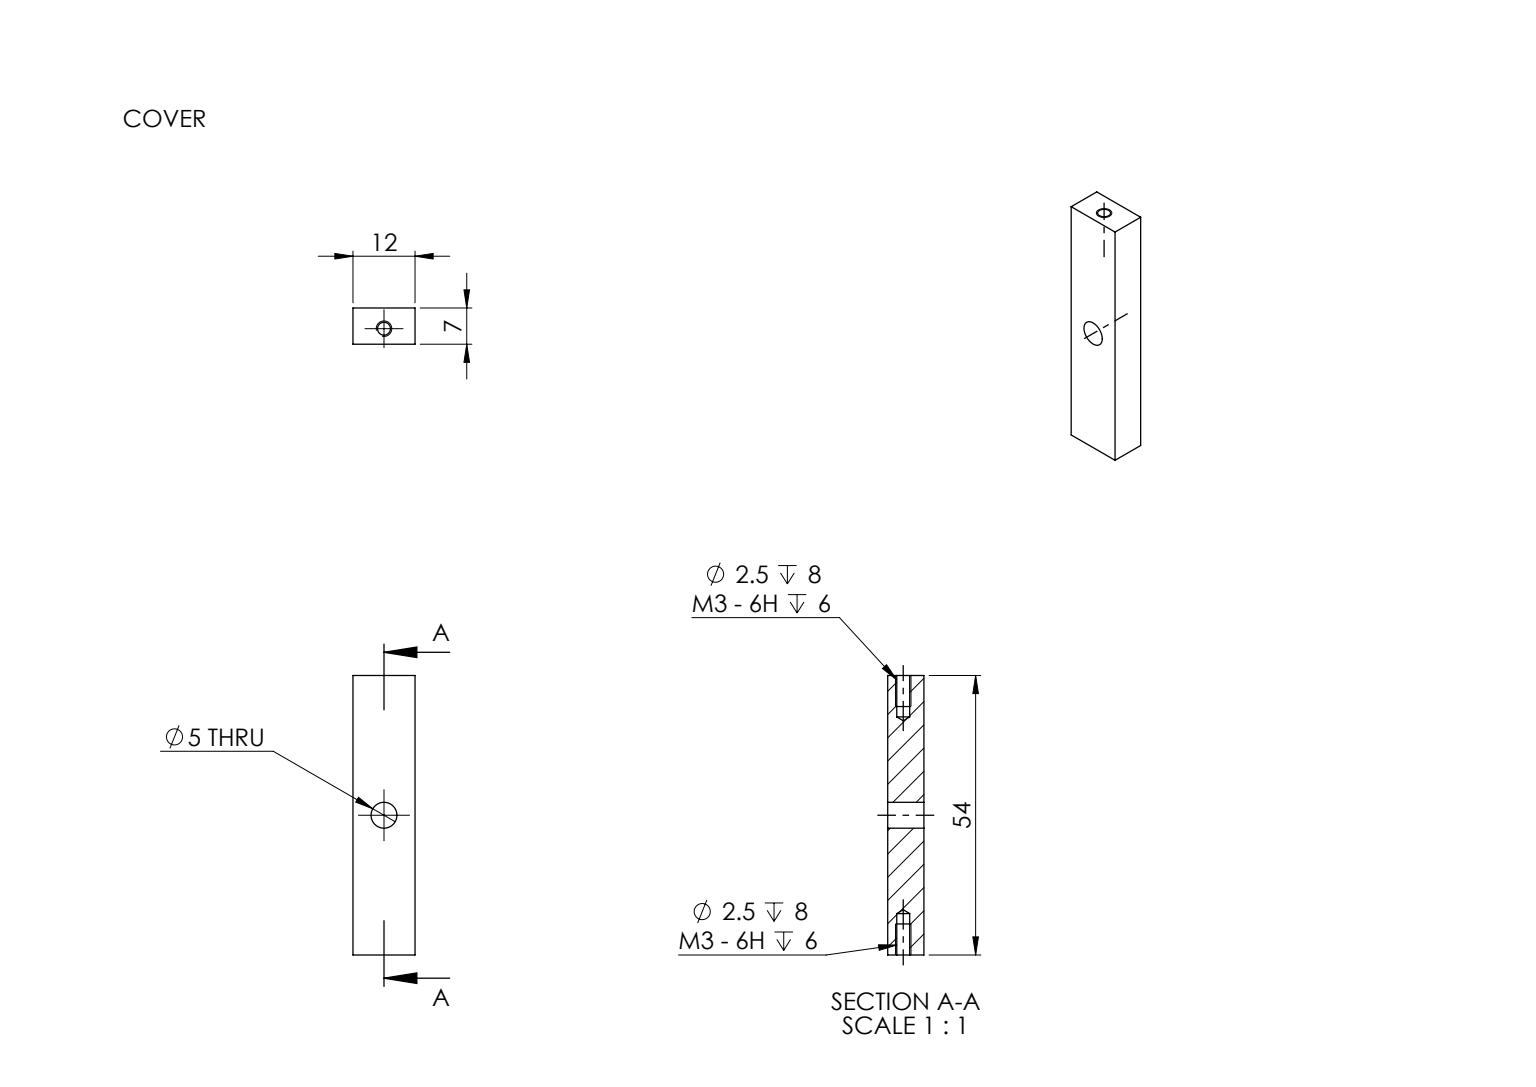
ISO-10303-21;
HEADER;
FILE_DESCRIPTION (('STEP AP214'),
    '1' );
FILE_NAME ('cover.step',
    '2026-10-03T18:28:46',
    ( '' ),
    ( '' ),
    'SwSTEP 2.0',
    'SolidWorks 2026',
    '' );
FILE_SCHEMA (( 'AUTOMOTIVE_DESIGN' ));
ENDSEC;

DATA;
#4=DIRECTION ( 'NONE',  ( 0.000000000000000000, 0.000000000000000000, 1.000000000000000000 ) ) ;
#12=PLANE ( 'NONE',  #9677 ) ;
#144=VERTEX_POINT ( 'NONE', #4838 ) ;
#200=CARTESIAN_POINT ( 'NONE',  ( 1.530808498934188612E-16, 18.99999999999999289, -1.249999999999997558 ) ) ;
#299=( NAMED_UNIT ( * ) SI_UNIT ( $, .STERADIAN. ) SOLID_ANGLE_UNIT ( ) );
#306=FACE_BOUND ( 'NONE', #5426, .T. ) ;
#314=ORIENTED_EDGE ( 'NONE', *, *, #8184, .T. ) ;
#318=DIRECTION ( 'NONE',  ( -0.000000000000000000, -1.000000000000000000, -0.000000000000000000 ) ) ;
#340=ADVANCED_FACE ( 'NONE', ( #9129 ), #3510, .F. ) ;
#376=VERTEX_POINT ( 'NONE', #586 ) ;
#381=DIRECTION ( 'NONE',  ( 1.000000000000000000, 0.000000000000000000, 0.000000000000000000 ) ) ;
#393=CARTESIAN_POINT ( 'NONE',  ( 5.999999999999999112, -27.00000000000000711, -4.000000000000000000 ) ) ;
#434=VECTOR ( 'NONE', #3012, 1000.000000000000000 ) ;
#442=CONICAL_SURFACE ( 'NONE', #7548, 1.249999999999997558, 1.029744258676650981 ) ;
#476=ORIENTED_EDGE ( 'NONE', *, *, #8711, .T. ) ;
#479=LINE ( 'NONE', #8439, #7690 ) ;
#491=LINE ( 'NONE', #2876, #2720 ) ;
#505=VERTEX_POINT ( 'NONE', #7751 ) ;
#514=AXIS2_PLACEMENT_3D ( 'NONE', #1323, #4706, #9556 ) ;
#518=LINE ( 'NONE', #5183, #846 ) ;
#555=ORIENTED_EDGE ( 'NONE', *, *, #4207, .T. ) ;
#586=CARTESIAN_POINT ( 'NONE',  ( 5.999999999999999112, -27.00000000000000711, 3.000000000000000000 ) ) ;
#608=AXIS2_PLACEMENT_3D ( 'NONE', #7258, #8118, #4082 ) ;
#678=CARTESIAN_POINT ( 'NONE',  ( -5.999999999999999112, 26.99999999999999289, 3.000000000000000000 ) ) ;
#712=EDGE_CURVE ( 'NONE', #980, #3093, #750, .T. ) ;
#736=ADVANCED_FACE ( 'NONE', ( #5713 ), #5223, .F. ) ;
#745=DIRECTION ( 'NONE',  ( 0.000000000000000000, 0.000000000000000000, -1.000000000000000000 ) ) ;
#750=LINE ( 'NONE', #3983, #6059 ) ;
#753=FACE_OUTER_BOUND ( 'NONE', #4033, .T. ) ;
#759=DIRECTION ( 'NONE',  ( 0.000000000000000000, 0.000000000000000000, 1.000000000000000000 ) ) ;
#766=VECTOR ( 'NONE', #8542, 1000.000000000000000 ) ;
#808=EDGE_CURVE ( 'NONE', #505, #2310, #6880, .T. ) ;
#822=CARTESIAN_POINT ( 'NONE',  ( 5.999999999999999112, -27.00000000000000711, 3.000000000000000000 ) ) ;
#823=LINE ( 'NONE', #9950, #1369 ) ;
#832=( NAMED_UNIT ( * ) SI_UNIT ( $, .STERADIAN. ) SOLID_ANGLE_UNIT ( ) );
#846=VECTOR ( 'NONE', #2165, 1000.000000000000000 ) ;
#851=DIRECTION ( 'NONE',  ( 1.000000000000000000, 0.000000000000000000, -0.000000000000000000 ) ) ;
#854=DIRECTION ( 'NONE',  ( -0.000000000000000000, -1.000000000000000000, -0.000000000000000000 ) ) ;
#856=ADVANCED_FACE ( 'NONE', ( #9639 ), #6825, .F. ) ;
#881=ORIENTED_EDGE ( 'NONE', *, *, #2871, .T. ) ;
#893=ORIENTED_EDGE ( 'NONE', *, *, #4207, .F. ) ;
#945=CARTESIAN_POINT ( 'NONE',  ( 5.999999999999999112, -27.00000000000000711, 3.000000000000000000 ) ) ;
#954=ORIENTED_EDGE ( 'NONE', *, *, #7254, .T. ) ;
#959=DIRECTION ( 'NONE',  ( 0.000000000000000000, 0.000000000000000000, 1.000000000000000000 ) ) ;
#968=DIRECTION ( 'NONE',  ( 0.000000000000000000, -0.000000000000000000, 1.000000000000000000 ) ) ;
#980=VERTEX_POINT ( 'NONE', #1783 ) ;
#999=AXIS2_PLACEMENT_3D ( 'NONE', #8960, #854, #1703 ) ;
#1002=LINE ( 'NONE', #6167, #3911 ) ;
#1048=DIRECTION ( 'NONE',  ( 0.000000000000000000, 0.000000000000000000, 1.000000000000000000 ) ) ;
#1072=CARTESIAN_POINT ( 'NONE',  ( 0.000000000000000000, 0.000000000000000000, 3.000000000000000000 ) ) ;
#1082=DIRECTION ( 'NONE',  ( 0.000000000000000000, 0.000000000000000000, 1.000000000000000000 ) ) ;
#1092=ORIENTED_EDGE ( 'NONE', *, *, #2254, .T. ) ;
#1117=ADVANCED_FACE ( 'NONE', ( #3941 ), #1519, .F. ) ;
#1213=FACE_OUTER_BOUND ( 'NONE', #9376, .T. ) ;
#1232=ADVANCED_FACE ( 'NONE', ( #4199 ), #9733, .F. ) ;
#1248=VERTEX_POINT ( 'NONE', #9686 ) ;
#1263=COLOUR_RGB ( '', 0.08235294, 0.09019608, 0.10196078) ;
#1265=ORIENTED_EDGE ( 'NONE', *, *, #6212, .T. ) ;
#1287=DIRECTION ( 'NONE',  ( -0.000000000000000000, 1.000000000000000000, -0.000000000000000000 ) ) ;
#1323=CARTESIAN_POINT ( 'NONE',  ( 0.000000000000000000, -27.00000000000000711, 0.000000000000000000 ) ) ;
#1331=EDGE_LOOP ( 'NONE', ( #6517, #9789, #7113 ) ) ;
#1334=LINE ( 'NONE', #10258, #2894 ) ;
#1349=VERTEX_POINT ( 'NONE', #6518 ) ;
#1351=AXIS2_PLACEMENT_3D ( 'NONE', #4874, #3979, #851 ) ;
#1359=ORIENTED_EDGE ( 'NONE', *, *, #6212, .F. ) ;
#1363=ADVANCED_FACE ( 'NONE', ( #2503, #753 ), #12, .F. ) ;
#1369=VECTOR ( 'NONE', #9141, 1000.000000000000000 ) ;
#1410=EDGE_LOOP ( 'NONE', ( #9527, #2908, #2491, #4743 ) ) ;
#1428=CARTESIAN_POINT ( 'NONE',  ( 1.530808498934183189E-16, 26.99999999999999289, -1.249999999999993339 ) ) ;
#1447=CARTESIAN_POINT ( 'NONE',  ( 0.000000000000000000, -19.00000000000000711, 0.000000000000000000 ) ) ;
#1448=CARTESIAN_POINT ( 'NONE',  ( 0.000000000000000000, 0.000000000000000000, -4.000000000000000000 ) ) ;
#1484=PRODUCT_DEFINITION_SHAPE ( 'NONE', 'NONE',  #7235 ) ;
#1488=DIRECTION ( 'NONE',  ( 0.000000000000000000, 0.000000000000000000, -1.000000000000000000 ) ) ;
#1517=EDGE_LOOP ( 'NONE', ( #6768, #8667, #1604, #8725 ) ) ;
#1519=CONICAL_SURFACE ( 'NONE', #7440, 1.249999999999997558, 1.029744258676650981 ) ;
#1523=CIRCLE ( 'NONE', #5067, 1.249999999999997558 ) ;
#1536=ORIENTED_EDGE ( 'NONE', *, *, #808, .F. ) ;
#1604=ORIENTED_EDGE ( 'NONE', *, *, #5366, .F. ) ;
#1610=CARTESIAN_POINT ( 'NONE',  ( 0.000000000000000000, 26.99999999999999289, 0.000000000000000000 ) ) ;
#1636=CARTESIAN_POINT ( 'NONE',  ( 0.000000000000000000, -19.00000000000000711, 0.000000000000000000 ) ) ;
#1648=CARTESIAN_POINT ( 'NONE',  ( -2.500000000000000000, 0.000000000000000000, -4.000000000000000000 ) ) ;
#1703=DIRECTION ( 'NONE',  ( 0.000000000000000000, 0.000000000000000000, -1.000000000000000000 ) ) ;
#1749=CARTESIAN_POINT ( 'NONE',  ( -5.999999999999999112, -27.00000000000000711, 3.000000000000000000 ) ) ;
#1760=CARTESIAN_POINT ( 'NONE',  ( -2.143395387092215042E-15, 18.24892422621553933, 0.000000000000000000 ) ) ;
#1776=STYLED_ITEM ( 'NONE', ( #2430 ), #4603 ) ;
#1783=CARTESIAN_POINT ( 'NONE',  ( 0.000000000000000000, -19.00000000000000711, -1.249999999999997558 ) ) ;
#1802=VERTEX_POINT ( 'NONE', #4484 ) ;
#1843=DIRECTION ( 'NONE',  ( -0.000000000000000000, -0.000000000000000000, -1.000000000000000000 ) ) ;
#1857=EDGE_LOOP ( 'NONE', ( #8302, #4110, #3466, #8986 ) ) ;
#1921=AXIS2_PLACEMENT_3D ( 'NONE', #4104, #7391, #9842 ) ;
#1938=SURFACE_SIDE_STYLE ('',( #5055 ) ) ;
#1940=DIRECTION ( 'NONE',  ( 1.049727191138616477E-16, 0.5150380749100571531, -0.8571673007021105573 ) ) ;
#1984=VERTEX_POINT ( 'NONE', #3956 ) ;
#2012=DIRECTION ( 'NONE',  ( 0.000000000000000000, 0.000000000000000000, -1.000000000000000000 ) ) ;
#2039=EDGE_CURVE ( 'NONE', #10462, #144, #1334, .T. ) ;
#2047=AXIS2_PLACEMENT_3D ( 'NONE', #4230, #7668, #6862 ) ;
#2059=ORIENTED_EDGE ( 'NONE', *, *, #712, .F. ) ;
#2087=DIRECTION ( 'NONE',  ( 0.000000000000000000, 0.000000000000000000, 1.000000000000000000 ) ) ;
#2092=ORIENTED_EDGE ( 'NONE', *, *, #8374, .F. ) ;
#2101=AXIS2_PLACEMENT_3D ( 'NONE', #7090, #5610, #4547 ) ;
#2107=ORIENTED_EDGE ( 'NONE', *, *, #2498, .F. ) ;
#2151=ORIENTED_EDGE ( 'NONE', *, *, #8374, .T. ) ;
#2165=DIRECTION ( 'NONE',  ( 0.000000000000000000, 0.5150380749100571531, 0.8571673007021105573 ) ) ;
#2185=EDGE_CURVE ( 'NONE', #2333, #7985, #10306, .T. ) ;
#2188=CYLINDRICAL_SURFACE ( 'NONE', #3728, 1.249999999999993339 ) ;
#2191=AXIS2_PLACEMENT_3D ( 'NONE', #9273, #3497, #2012 ) ;
#2198=AXIS2_PLACEMENT_3D ( 'NONE', #6512, #3925, #1488 ) ;
#2204=VECTOR ( 'NONE', #5118, 1000.000000000000000 ) ;
#2216=ORIENTED_EDGE ( 'NONE', *, *, #7634, .T. ) ;
#2254=EDGE_CURVE ( 'NONE', #2333, #3169, #4079, .T. ) ;
#2291=ADVANCED_FACE ( 'NONE', ( #10464 ), #5710, .F. ) ;
#2310=VERTEX_POINT ( 'NONE', #1648 ) ;
#2332=CARTESIAN_POINT ( 'NONE',  ( 5.999999999999999112, 26.99999999999999289, -4.000000000000000000 ) ) ;
#2333=VERTEX_POINT ( 'NONE', #9816 ) ;
#2368=CIRCLE ( 'NONE', #2191, 1.249999999999988898 ) ;
#2382=AXIS2_PLACEMENT_3D ( 'NONE', #945, #5065, #1048 ) ;
#2430=PRESENTATION_STYLE_ASSIGNMENT (( #9052 ) ) ;
#2450=DIRECTION ( 'NONE',  ( -0.000000000000000000, -1.000000000000000000, -0.000000000000000000 ) ) ;
#2464=ADVANCED_FACE ( 'NONE', ( #4525 ), #8276, .F. ) ;
#2471=ORIENTED_EDGE ( 'NONE', *, *, #4014, .F. ) ;
#2491=ORIENTED_EDGE ( 'NONE', *, *, #9814, .T. ) ;
#2498=EDGE_CURVE ( 'NONE', #1349, #2589, #1002, .T. ) ;
#2503=FACE_BOUND ( 'NONE', #5490, .T. ) ;
#2529=FILL_AREA_STYLE_COLOUR ( '', #1263 ) ;
#2585=EDGE_LOOP ( 'NONE', ( #7497, #6215 ) ) ;
#2589=VERTEX_POINT ( 'NONE', #3684 ) ;
#2638=CARTESIAN_POINT ( 'NONE',  ( 1.530808498934183189E-16, -27.00000000000000711, 1.249999999999993339 ) ) ;
#2639=ORIENTED_EDGE ( 'NONE', *, *, #5366, .T. ) ;
#2673=EDGE_CURVE ( 'NONE', #376, #8882, #4052, .T. ) ;
#2684=ORIENTED_EDGE ( 'NONE', *, *, #6082, .F. ) ;
#2699=CARTESIAN_POINT ( 'NONE',  ( 1.530808498934180724E-16, 26.99999999999999289, -1.249999999999988898 ) ) ;
#2720=VECTOR ( 'NONE', #5313, 1000.000000000000000 ) ;
#2732=( NAMED_UNIT ( * ) PLANE_ANGLE_UNIT ( ) SI_UNIT ( $, .RADIAN. ) );
#2738=VERTEX_POINT ( 'NONE', #4684 ) ;
#2765=DIRECTION ( 'NONE',  ( 0.000000000000000000, 0.000000000000000000, 1.000000000000000000 ) ) ;
#2782=( LENGTH_UNIT ( ) NAMED_UNIT ( * ) SI_UNIT ( .MILLI., .METRE. ) );
#2827=FACE_OUTER_BOUND ( 'NONE', #1857, .T. ) ;
#2829=LINE ( 'NONE', #393, #4246 ) ;
#2851=CARTESIAN_POINT ( 'NONE',  ( 0.000000000000000000, 18.99999999999999289, 0.000000000000000000 ) ) ;
#2871=EDGE_CURVE ( 'NONE', #2310, #2589, #6449, .T. ) ;
#2876=CARTESIAN_POINT ( 'NONE',  ( 5.999999999999999112, -27.00000000000000711, 3.000000000000000000 ) ) ;
#2889=VECTOR ( 'NONE', #6206, 1000.000000000000000 ) ;
#2894=VECTOR ( 'NONE', #9353, 1000.000000000000000 ) ;
#2908=ORIENTED_EDGE ( 'NONE', *, *, #10395, .T. ) ;
#2936=DIRECTION ( 'NONE',  ( 1.000000000000000000, -0.000000000000000000, -0.000000000000000000 ) ) ;
#2937=EDGE_CURVE ( 'NONE', #9930, #8882, #2829, .T. ) ;
#2975=CYLINDRICAL_SURFACE ( 'NONE', #514, 1.249999999999993339 ) ;
#3012=DIRECTION ( 'NONE',  ( -0.000000000000000000, -1.000000000000000000, -0.000000000000000000 ) ) ;
#3013=DIRECTION ( 'NONE',  ( 0.000000000000000000, 0.000000000000000000, 1.000000000000000000 ) ) ;
#3067=ORIENTED_EDGE ( 'NONE', *, *, #6295, .F. ) ;
#3085=CARTESIAN_POINT ( 'NONE',  ( -5.999999999999999112, -27.00000000000000711, -4.000000000000000000 ) ) ;
#3093=VERTEX_POINT ( 'NONE', #6105 ) ;
#3165=( NAMED_UNIT ( * ) PLANE_ANGLE_UNIT ( ) SI_UNIT ( $, .RADIAN. ) );
#3169=VERTEX_POINT ( 'NONE', #4725 ) ;
#3236=FACE_OUTER_BOUND ( 'NONE', #4534, .T. ) ;
#3242=DIRECTION ( 'NONE',  ( 0.000000000000000000, -1.000000000000000000, 0.000000000000000000 ) ) ;
#3246=PRODUCT_CONTEXT ( 'NONE', #3297, 'mechanical' ) ;
#3254=CARTESIAN_POINT ( 'NONE',  ( -5.999999999999999112, -27.00000000000000711, 3.000000000000000000 ) ) ;
#3262=EDGE_LOOP ( 'NONE', ( #4954, #10176, #7125, #4590 ) ) ;
#3297=APPLICATION_CONTEXT ( 'automotive_design' ) ;
#3321=ADVANCED_FACE ( 'NONE', ( #3774 ), #442, .F. ) ;
#3466=ORIENTED_EDGE ( 'NONE', *, *, #2185, .T. ) ;
#3496=EDGE_LOOP ( 'NONE', ( #314, #2151, #5786, #2639 ) ) ;
#3497=DIRECTION ( 'NONE',  ( -0.000000000000000000, -1.000000000000000000, -0.000000000000000000 ) ) ;
#3510=CYLINDRICAL_SURFACE ( 'NONE', #8258, 1.249999999999993339 ) ;
#3629=ORIENTED_EDGE ( 'NONE', *, *, #6933, .T. ) ;
#3651=AXIS2_PLACEMENT_3D ( 'NONE', #1072, #2765, #381 ) ;
#3653=DIRECTION ( 'NONE',  ( -0.000000000000000000, -0.000000000000000000, -1.000000000000000000 ) ) ;
#3684=CARTESIAN_POINT ( 'NONE',  ( 2.500000000000000000, 3.061616997868383141E-16, -4.000000000000000000 ) ) ;
#3692=ORIENTED_EDGE ( 'NONE', *, *, #7915, .F. ) ;
#3718=AXIS2_PLACEMENT_3D ( 'NONE', #2851, #5387, #3013 ) ;
#3720=STYLED_ITEM ( 'NONE', ( #7505 ), #4735 ) ;
#3728=AXIS2_PLACEMENT_3D ( 'NONE', #6041, #1287, #2087 ) ;
#3751=CARTESIAN_POINT ( 'NONE',  ( 0.000000000000000000, -27.00000000000000711, 0.000000000000000000 ) ) ;
#3774=FACE_OUTER_BOUND ( 'NONE', #1331, .T. ) ;
#3857=DIRECTION ( 'NONE',  ( -0.000000000000000000, -1.000000000000000000, -0.000000000000000000 ) ) ;
#3890=ORIENTED_EDGE ( 'NONE', *, *, #9814, .F. ) ;
#3911=VECTOR ( 'NONE', #4476, 1000.000000000000000 ) ;
#3925=DIRECTION ( 'NONE',  ( -0.000000000000000000, -1.000000000000000000, -0.000000000000000000 ) ) ;
#3941=FACE_OUTER_BOUND ( 'NONE', #7990, .T. ) ;
#3942=DIRECTION ( 'NONE',  ( -0.000000000000000000, -0.000000000000000000, -1.000000000000000000 ) ) ;
#3956=CARTESIAN_POINT ( 'NONE',  ( -2.143395387092215042E-15, -18.24892422621555355, 0.000000000000000000 ) ) ;
#3968=CARTESIAN_POINT ( 'NONE',  ( -5.999999999999999112, 26.99999999999999289, 3.000000000000000000 ) ) ;
#3979=DIRECTION ( 'NONE',  ( 0.000000000000000000, -0.000000000000000000, 1.000000000000000000 ) ) ;
#3983=CARTESIAN_POINT ( 'NONE',  ( 0.000000000000000000, -27.00000000000000711, -1.249999999999993339 ) ) ;
#3998=AXIS2_PLACEMENT_3D ( 'NONE', #1610, #8132, #759 ) ;
#4003=UNCERTAINTY_MEASURE_WITH_UNIT (LENGTH_MEASURE( 1.000000000000000082E-05 ), #5649, 'distance_accuracy_value', 'NONE');
#4014=EDGE_CURVE ( 'NONE', #8882, #10462, #8279, .T. ) ;
#4019=ORIENTED_EDGE ( 'NONE', *, *, #4025, .T. ) ;
#4025=EDGE_CURVE ( 'NONE', #3169, #2333, #1523, .T. ) ;
#4033=EDGE_LOOP ( 'NONE', ( #8278, #7652, #2092, #9801 ) ) ;
#4052=LINE ( 'NONE', #822, #4927 ) ;
#4063=( NAMED_UNIT ( * ) SI_UNIT ( $, .STERADIAN. ) SOLID_ANGLE_UNIT ( ) );
#4079=CIRCLE ( 'NONE', #10360, 1.249999999999997558 ) ;
#4082=DIRECTION ( 'NONE',  ( 1.000000000000000000, 0.000000000000000000, 0.000000000000000000 ) ) ;
#4104=CARTESIAN_POINT ( 'NONE',  ( 0.000000000000000000, 26.99999999999999289, 0.000000000000000000 ) ) ;
#4108=DIRECTION ( 'NONE',  ( 1.000000000000000000, 0.000000000000000000, 0.000000000000000000 ) ) ;
#4110=ORIENTED_EDGE ( 'NONE', *, *, #2254, .F. ) ;
#4115=VERTEX_POINT ( 'NONE', #2699 ) ;
#4140=EDGE_CURVE ( 'NONE', #980, #2738, #5397, .T. ) ;
#4171=LINE ( 'NONE', #2638, #2204 ) ;
#4188=ORIENTED_EDGE ( 'NONE', *, *, #2871, .F. ) ;
#4199=FACE_OUTER_BOUND ( 'NONE', #7216, .T. ) ;
#4207=EDGE_CURVE ( 'NONE', #9761, #3093, #2368, .T. ) ;
#4214=FILL_AREA_STYLE ('',( #2529 ) ) ;
#4230=CARTESIAN_POINT ( 'NONE',  ( 5.999999999999999112, -27.00000000000000711, 3.000000000000000000 ) ) ;
#4234=DIRECTION ( 'NONE',  ( 0.000000000000000000, 1.000000000000000000, 0.000000000000000000 ) ) ;
#4246=VECTOR ( 'NONE', #2936, 1000.000000000000000 ) ;
#4259=SURFACE_STYLE_USAGE ( .BOTH. , #1938 ) ;
#4284=CARTESIAN_POINT ( 'NONE',  ( 0.000000000000000000, -19.00000000000000711, 0.000000000000000000 ) ) ;
#4347=DIRECTION ( 'NONE',  ( -0.000000000000000000, 1.000000000000000000, -0.000000000000000000 ) ) ;
#4398=PLANE ( 'NONE',  #9591 ) ;
#4444=VECTOR ( 'NONE', #4863, 1000.000000000000000 ) ;
#4472=( GEOMETRIC_REPRESENTATION_CONTEXT ( 3 ) GLOBAL_UNCERTAINTY_ASSIGNED_CONTEXT ( ( #8527 ) ) GLOBAL_UNIT_ASSIGNED_CONTEXT ( ( #8220, #8262, #832 ) ) REPRESENTATION_CONTEXT ( 'NONE', 'WORKASPACE' ) );
#4476=DIRECTION ( 'NONE',  ( -0.000000000000000000, -0.000000000000000000, -1.000000000000000000 ) ) ;
#4484=CARTESIAN_POINT ( 'NONE',  ( 5.999999999999999112, 26.99999999999999289, 3.000000000000000000 ) ) ;
#4525=FACE_OUTER_BOUND ( 'NONE', #3262, .T. ) ;
#4534=EDGE_LOOP ( 'NONE', ( #2471, #7142, #1359, #7756 ) ) ;
#4547=DIRECTION ( 'NONE',  ( 1.000000000000000000, 0.000000000000000000, 0.000000000000000000 ) ) ;
#4557=MECHANICAL_DESIGN_GEOMETRIC_PRESENTATION_REPRESENTATION('',(#3720),#5076);
#4576=AXIS2_PLACEMENT_3D ( 'NONE', #1749, #9716, #745 ) ;
#4590=ORIENTED_EDGE ( 'NONE', *, *, #2673, .T. ) ;
#4603=ADVANCED_BREP_SHAPE_REPRESENTATION ( '', ( #4735, #2101 ), #4472 ) ;
#4673=DIRECTION ( 'NONE',  ( 0.000000000000000000, 0.000000000000000000, -1.000000000000000000 ) ) ;
#4684=CARTESIAN_POINT ( 'NONE',  ( 1.530808498934188612E-16, -19.00000000000000711, 1.249999999999997558 ) ) ;
#4706=DIRECTION ( 'NONE',  ( -0.000000000000000000, -1.000000000000000000, -0.000000000000000000 ) ) ;
#4725=CARTESIAN_POINT ( 'NONE',  ( 1.530808498934188612E-16, 18.99999999999999289, -1.249999999999997558 ) ) ;
#4731=PRODUCT_DEFINITION_CONTEXT ( 'detailed design', #9259, 'design' ) ;
#4735=MANIFOLD_SOLID_BREP ( 'M3 Tapped Hole2', #7609 ) ;
#4743=ORIENTED_EDGE ( 'NONE', *, *, #2185, .F. ) ;
#4781=SHAPE_DEFINITION_REPRESENTATION ( #1484, #7954 ) ;
#4832=VECTOR ( 'NONE', #7782, 1000.000000000000000 ) ;
#4838=CARTESIAN_POINT ( 'NONE',  ( -5.999999999999999112, 26.99999999999999289, -4.000000000000000000 ) ) ;
#4840=CARTESIAN_POINT ( 'NONE',  ( 0.000000000000000000, 0.000000000000000000, 3.000000000000000000 ) ) ;
#4847=ORIENTED_EDGE ( 'NONE', *, *, #7915, .T. ) ;
#4863=DIRECTION ( 'NONE',  ( -0.000000000000000000, -0.000000000000000000, -1.000000000000000000 ) ) ;
#4874=CARTESIAN_POINT ( 'NONE',  ( 0.000000000000000000, 0.000000000000000000, -4.000000000000000000 ) ) ;
#4910=EDGE_LOOP ( 'NONE', ( #881, #476 ) ) ;
#4927=VECTOR ( 'NONE', #6324, 1000.000000000000000 ) ;
#4931=PLANE ( 'NONE',  #1351 ) ;
#4954=ORIENTED_EDGE ( 'NONE', *, *, #4014, .T. ) ;
#4962=ORIENTED_EDGE ( 'NONE', *, *, #808, .T. ) ;
#4963=VECTOR ( 'NONE', #1940, 1000.000000000000000 ) ;
#4965=EDGE_CURVE ( 'NONE', #1248, #9930, #6376, .T. ) ;
#4981=CARTESIAN_POINT ( 'NONE',  ( 5.999999999999999112, -27.00000000000000711, -4.000000000000000000 ) ) ;
#5017=ADVANCED_FACE ( 'NONE', ( #5350 ), #2975, .F. ) ;
#5055=SURFACE_STYLE_FILL_AREA ( #9145 ) ;
#5065=DIRECTION ( 'NONE',  ( 0.000000000000000000, 1.000000000000000000, -0.000000000000000000 ) ) ;
#5067=AXIS2_PLACEMENT_3D ( 'NONE', #9016, #9664, #959 ) ;
#5076=( GEOMETRIC_REPRESENTATION_CONTEXT ( 3 ) GLOBAL_UNCERTAINTY_ASSIGNED_CONTEXT ( ( #6065 ) ) GLOBAL_UNIT_ASSIGNED_CONTEXT ( ( #2782, #2732, #299 ) ) REPRESENTATION_CONTEXT ( 'NONE', 'WORKASPACE' ) );
#5091=AXIS2_PLACEMENT_3D ( 'NONE', #1448, #6260, #5574 ) ;
#5118=DIRECTION ( 'NONE',  ( -0.000000000000000000, -1.000000000000000000, -0.000000000000000000 ) ) ;
#5176=CIRCLE ( 'NONE', #608, 2.500000000000000000 ) ;
#5183=CARTESIAN_POINT ( 'NONE',  ( 0.000000000000000000, 18.99999999999999289, 1.249999999999997558 ) ) ;
#5196=FACE_OUTER_BOUND ( 'NONE', #3496, .T. ) ;
#5223=CONICAL_SURFACE ( 'NONE', #999, 1.249999999999997558, 1.029744258676650981 ) ;
#5252=VECTOR ( 'NONE', #3942, 1000.000000000000000 ) ;
#5276=ADVANCED_FACE ( 'NONE', ( #2827 ), #2188, .F. ) ;
#5288=CARTESIAN_POINT ( 'NONE',  ( 0.000000000000000000, -19.00000000000000711, -1.249999999999997558 ) ) ;
#5313=DIRECTION ( 'NONE',  ( 1.000000000000000000, -0.000000000000000000, -0.000000000000000000 ) ) ;
#5350=FACE_OUTER_BOUND ( 'NONE', #9570, .T. ) ;
#5366=EDGE_CURVE ( 'NONE', #1248, #376, #491, .T. ) ;
#5374=LINE ( 'NONE', #8614, #7288 ) ;
#5387=DIRECTION ( 'NONE',  ( -0.000000000000000000, 1.000000000000000000, -0.000000000000000000 ) ) ;
#5397=CIRCLE ( 'NONE', #6241, 1.249999999999997558 ) ;
#5426=EDGE_LOOP ( 'NONE', ( #7263, #893 ) ) ;
#5490=EDGE_LOOP ( 'NONE', ( #5867, #3890 ) ) ;
#5508=FACE_OUTER_BOUND ( 'NONE', #5758, .T. ) ;
#5527=EDGE_CURVE ( 'NONE', #1984, #2738, #6888, .T. ) ;
#5549=LINE ( 'NONE', #3968, #4444 ) ;
#5574=DIRECTION ( 'NONE',  ( 1.000000000000000000, 0.000000000000000000, 0.000000000000000000 ) ) ;
#5590=CARTESIAN_POINT ( 'NONE',  ( 0.000000000000000000, 0.000000000000000000, 3.000000000000000000 ) ) ;
#5610=DIRECTION ( 'NONE',  ( 0.000000000000000000, 0.000000000000000000, 1.000000000000000000 ) ) ;
#5649=( LENGTH_UNIT ( ) NAMED_UNIT ( * ) SI_UNIT ( .MILLI., .METRE. ) );
#5710=PLANE ( 'NONE',  #4576 ) ;
#5713=FACE_OUTER_BOUND ( 'NONE', #7414, .T. ) ;
#5716=DIRECTION ( 'NONE',  ( 0.000000000000000000, -0.000000000000000000, -1.000000000000000000 ) ) ;
#5758=EDGE_LOOP ( 'NONE', ( #3692, #8102, #6558, #9293 ) ) ;
#5786=ORIENTED_EDGE ( 'NONE', *, *, #10280, .T. ) ;
#5799=SURFACE_STYLE_FILL_AREA ( #4214 ) ;
#5867=ORIENTED_EDGE ( 'NONE', *, *, #6749, .F. ) ;
#5997=FILL_AREA_STYLE_COLOUR ( '', #8308 ) ;
#6041=CARTESIAN_POINT ( 'NONE',  ( 0.000000000000000000, 26.99999999999999289, 0.000000000000000000 ) ) ;
#6059=VECTOR ( 'NONE', #2450, 1000.000000000000000 ) ;
#6065=UNCERTAINTY_MEASURE_WITH_UNIT (LENGTH_MEASURE( 1.000000000000000082E-05 ), #2782, 'distance_accuracy_value', 'NONE');
#6082=EDGE_CURVE ( 'NONE', #1984, #980, #9436, .T. ) ;
#6086=CARTESIAN_POINT ( 'NONE',  ( 1.530808498934188612E-16, -19.00000000000000711, 1.249999999999997558 ) ) ;
#6103=AXIS2_PLACEMENT_3D ( 'NONE', #9140, #1082, #4108 ) ;
#6105=CARTESIAN_POINT ( 'NONE',  ( 0.000000000000000000, -27.00000000000000711, -1.249999999999988898 ) ) ;
#6159=CARTESIAN_POINT ( 'NONE',  ( 0.000000000000000000, 18.99999999999999289, 0.000000000000000000 ) ) ;
#6167=CARTESIAN_POINT ( 'NONE',  ( 2.500000000000000000, 3.061616997868383141E-16, 3.000000000000000000 ) ) ;
#6172=( GEOMETRIC_REPRESENTATION_CONTEXT ( 3 ) GLOBAL_UNCERTAINTY_ASSIGNED_CONTEXT ( ( #4003 ) ) GLOBAL_UNIT_ASSIGNED_CONTEXT ( ( #5649, #3165, #4063 ) ) REPRESENTATION_CONTEXT ( 'NONE', 'WORKASPACE' ) );
#6174=ORIENTED_EDGE ( 'NONE', *, *, #9678, .F. ) ;
#6206=DIRECTION ( 'NONE',  ( -0.000000000000000000, 1.000000000000000000, -0.000000000000000000 ) ) ;
#6212=EDGE_CURVE ( 'NONE', #144, #9930, #8894, .T. ) ;
#6215=ORIENTED_EDGE ( 'NONE', *, *, #7254, .F. ) ;
#6241=AXIS2_PLACEMENT_3D ( 'NONE', #4284, #318, #9975 ) ;
#6260=DIRECTION ( 'NONE',  ( 0.000000000000000000, 0.000000000000000000, 1.000000000000000000 ) ) ;
#6295=EDGE_CURVE ( 'NONE', #2738, #980, #8719, .T. ) ;
#6323=CIRCLE ( 'NONE', #10415, 1.249999999999988898 ) ;
#6324=DIRECTION ( 'NONE',  ( -0.000000000000000000, -0.000000000000000000, -1.000000000000000000 ) ) ;
#6375=DIRECTION ( 'NONE',  ( 0.000000000000000000, 0.000000000000000000, 1.000000000000000000 ) ) ;
#6376=LINE ( 'NONE', #3254, #5252 ) ;
#6403=FACE_BOUND ( 'NONE', #4910, .T. ) ;
#6408=ORIENTED_EDGE ( 'NONE', *, *, #8711, .F. ) ;
#6449=CIRCLE ( 'NONE', #6103, 2.500000000000000000 ) ;
#6479=CIRCLE ( 'NONE', #1921, 1.249999999999988898 ) ;
#6512=CARTESIAN_POINT ( 'NONE',  ( 0.000000000000000000, -27.00000000000000711, 0.000000000000000000 ) ) ;
#6517=ORIENTED_EDGE ( 'NONE', *, *, #5527, .F. ) ;
#6518=CARTESIAN_POINT ( 'NONE',  ( 2.500000000000000000, 3.061616997868383141E-16, 3.000000000000000000 ) ) ;
#6533=DIRECTION ( 'NONE',  ( -1.000000000000000000, 0.000000000000000000, 0.000000000000000000 ) ) ;
#6537=CARTESIAN_POINT ( 'NONE',  ( 1.530808498934180724E-16, -27.00000000000000711, 1.249999999999988898 ) ) ;
#6549=SHAPE_REPRESENTATION_RELATIONSHIP ( 'NONE' , 'NONE' ,  #7954, #4603 ) ;
#6558=ORIENTED_EDGE ( 'NONE', *, *, #712, .T. ) ;
#6749=EDGE_CURVE ( 'NONE', #7985, #4115, #7885, .T. ) ;
#6768=ORIENTED_EDGE ( 'NONE', *, *, #2937, .T. ) ;
#6825=CYLINDRICAL_SURFACE ( 'NONE', #8787, 2.500000000000000000 ) ;
#6858=CIRCLE ( 'NONE', #3651, 2.500000000000000000 ) ;
#6862=DIRECTION ( 'NONE',  ( 0.000000000000000000, 0.000000000000000000, 1.000000000000000000 ) ) ;
#6880=LINE ( 'NONE', #9275, #7940 ) ;
#6888=LINE ( 'NONE', #6086, #766 ) ;
#6933=EDGE_CURVE ( 'NONE', #505, #1349, #6858, .T. ) ;
#6967=ORIENTED_EDGE ( 'NONE', *, *, #5527, .T. ) ;
#7012=EDGE_LOOP ( 'NONE', ( #3629, #9462, #4188, #1536 ) ) ;
#7024=AXIS2_PLACEMENT_3D ( 'NONE', #1636, #9595, #7889 ) ;
#7063=ADVANCED_FACE ( 'NONE', ( #5196, #8441 ), #4398, .T. ) ;
#7074=ORIENTED_EDGE ( 'NONE', *, *, #7634, .F. ) ;
#7090=CARTESIAN_POINT ( 'NONE',  ( 0.000000000000000000, 0.000000000000000000, 0.000000000000000000 ) ) ;
#7091=VECTOR ( 'NONE', #4234, 1000.000000000000000 ) ;
#7113=ORIENTED_EDGE ( 'NONE', *, *, #4140, .T. ) ;
#7125=ORIENTED_EDGE ( 'NONE', *, *, #8184, .F. ) ;
#7142=ORIENTED_EDGE ( 'NONE', *, *, #2937, .F. ) ;
#7168=DIRECTION ( 'NONE',  ( -0.000000000000000000, 1.000000000000000000, -0.000000000000000000 ) ) ;
#7216=EDGE_LOOP ( 'NONE', ( #2107, #954, #4962, #6408 ) ) ;
#7235=PRODUCT_DEFINITION ( 'UNKNOWN', '', #9232, #4731 ) ;
#7247=ORIENTED_EDGE ( 'NONE', *, *, #9678, .T. ) ;
#7254=EDGE_CURVE ( 'NONE', #1349, #505, #5176, .T. ) ;
#7258=CARTESIAN_POINT ( 'NONE',  ( 0.000000000000000000, 0.000000000000000000, 3.000000000000000000 ) ) ;
#7263=ORIENTED_EDGE ( 'NONE', *, *, #9009, .F. ) ;
#7288=VECTOR ( 'NONE', #8884, 1000.000000000000000 ) ;
#7291=ADVANCED_FACE ( 'NONE', ( #5508 ), #8958, .F. ) ;
#7312=ADVANCED_FACE ( 'NONE', ( #3236, #6403 ), #4931, .F. ) ;
#7391=DIRECTION ( 'NONE',  ( -0.000000000000000000, 1.000000000000000000, -0.000000000000000000 ) ) ;
#7414=EDGE_LOOP ( 'NONE', ( #2684, #6967, #10456 ) ) ;
#7440=AXIS2_PLACEMENT_3D ( 'NONE', #6159, #7168, #6375 ) ;
#7455=LINE ( 'NONE', #200, #4963 ) ;
#7497=ORIENTED_EDGE ( 'NONE', *, *, #6933, .F. ) ;
#7505=PRESENTATION_STYLE_ASSIGNMENT (( #4259 ) ) ;
#7548=AXIS2_PLACEMENT_3D ( 'NONE', #1447, #9571, #4673 ) ;
#7587=ADVANCED_FACE ( 'NONE', ( #1213 ), #10333, .F. ) ;
#7588=DIRECTION ( 'NONE',  ( 0.000000000000000000, 0.000000000000000000, 1.000000000000000000 ) ) ;
#7609=CLOSED_SHELL ( 'NONE', ( #5017, #736, #340, #7587, #856, #7063, #7312, #2464, #1363, #2291, #7913, #1232, #1117, #5276, #3321, #7291 ) ) ;
#7634=EDGE_CURVE ( 'NONE', #10224, #2333, #518, .T. ) ;
#7645=CARTESIAN_POINT ( 'NONE',  ( 0.000000000000000000, 0.000000000000000000, 3.000000000000000000 ) ) ;
#7652=ORIENTED_EDGE ( 'NONE', *, *, #9365, .F. ) ;
#7668=DIRECTION ( 'NONE',  ( -1.000000000000000000, 0.000000000000000000, 0.000000000000000000 ) ) ;
#7688=DIRECTION ( 'NONE',  ( -0.000000000000000000, -0.000000000000000000, -1.000000000000000000 ) ) ;
#7690=VECTOR ( 'NONE', #9233, 1000.000000000000000 ) ;
#7731=EDGE_LOOP ( 'NONE', ( #1265, #9539, #9108, #7819 ) ) ;
#7751=CARTESIAN_POINT ( 'NONE',  ( -2.500000000000000000, 0.000000000000000000, 3.000000000000000000 ) ) ;
#7756=ORIENTED_EDGE ( 'NONE', *, *, #2039, .F. ) ;
#7779=VERTEX_POINT ( 'NONE', #678 ) ;
#7782=DIRECTION ( 'NONE',  ( 0.000000000000000000, -0.5150380749100571531, -0.8571673007021105573 ) ) ;
#7819=ORIENTED_EDGE ( 'NONE', *, *, #9365, .T. ) ;
#7848=DIRECTION ( 'NONE',  ( 1.000000000000000000, 0.000000000000000000, -0.000000000000000000 ) ) ;
#7885=CIRCLE ( 'NONE', #3998, 1.249999999999988898 ) ;
#7889=DIRECTION ( 'NONE',  ( 0.000000000000000000, 0.000000000000000000, -1.000000000000000000 ) ) ;
#7913=ADVANCED_FACE ( 'NONE', ( #306, #8944 ), #8317, .F. ) ;
#7915=EDGE_CURVE ( 'NONE', #2738, #9761, #4171, .T. ) ;
#7940=VECTOR ( 'NONE', #7688, 1000.000000000000000 ) ;
#7954=SHAPE_REPRESENTATION ( 'cover', ( #2101 ), #4472 ) ;
#7985=VERTEX_POINT ( 'NONE', #9055 ) ;
#7990=EDGE_LOOP ( 'NONE', ( #6174, #2216, #1092 ) ) ;
#7995=EDGE_CURVE ( 'NONE', #1802, #10462, #9107, .T. ) ;
#8010=DIRECTION ( 'NONE',  ( -0.000000000000000000, 1.000000000000000000, -0.000000000000000000 ) ) ;
#8051=SURFACE_SIDE_STYLE ('',( #5799 ) ) ;
#8102=ORIENTED_EDGE ( 'NONE', *, *, #4140, .F. ) ;
#8118=DIRECTION ( 'NONE',  ( 0.000000000000000000, 0.000000000000000000, 1.000000000000000000 ) ) ;
#8132=DIRECTION ( 'NONE',  ( -0.000000000000000000, 1.000000000000000000, -0.000000000000000000 ) ) ;
#8141=VECTOR ( 'NONE', #1843, 1000.000000000000000 ) ;
#8184=EDGE_CURVE ( 'NONE', #376, #1802, #5374, .T. ) ;
#8220=( LENGTH_UNIT ( ) NAMED_UNIT ( * ) SI_UNIT ( .MILLI., .METRE. ) );
#8258=AXIS2_PLACEMENT_3D ( 'NONE', #9989, #4347, #7588 ) ;
#8262=( NAMED_UNIT ( * ) PLANE_ANGLE_UNIT ( ) SI_UNIT ( $, .RADIAN. ) );
#8276=PLANE ( 'NONE',  #2047 ) ;
#8278=ORIENTED_EDGE ( 'NONE', *, *, #2039, .T. ) ;
#8279=LINE ( 'NONE', #4981, #7091 ) ;
#8302=ORIENTED_EDGE ( 'NONE', *, *, #10395, .F. ) ;
#8308=COLOUR_RGB ( '', 0.08235294, 0.09019608, 0.10196078) ;
#8317=PLANE ( 'NONE',  #2382 ) ;
#8374=EDGE_CURVE ( 'NONE', #1802, #7779, #823, .T. ) ;
#8439=CARTESIAN_POINT ( 'NONE',  ( -5.999999999999999112, -27.00000000000000711, 3.000000000000000000 ) ) ;
#8441=FACE_BOUND ( 'NONE', #2585, .T. ) ;
#8527=UNCERTAINTY_MEASURE_WITH_UNIT (LENGTH_MEASURE( 1.000000000000000082E-05 ), #8220, 'distance_accuracy_value', 'NONE');
#8542=DIRECTION ( 'NONE',  ( 1.049727191138616477E-16, -0.5150380749100571531, 0.8571673007021105573 ) ) ;
#8614=CARTESIAN_POINT ( 'NONE',  ( 5.999999999999999112, -27.00000000000000711, 3.000000000000000000 ) ) ;
#8667=ORIENTED_EDGE ( 'NONE', *, *, #2673, .F. ) ;
#8711=EDGE_CURVE ( 'NONE', #2589, #2310, #10011, .T. ) ;
#8719=CIRCLE ( 'NONE', #7024, 1.249999999999997558 ) ;
#8725=ORIENTED_EDGE ( 'NONE', *, *, #4965, .T. ) ;
#8787=AXIS2_PLACEMENT_3D ( 'NONE', #5590, #3653, #10322 ) ;
#8882=VERTEX_POINT ( 'NONE', #8976 ) ;
#8884=DIRECTION ( 'NONE',  ( 0.000000000000000000, 1.000000000000000000, 0.000000000000000000 ) ) ;
#8894=LINE ( 'NONE', #9646, #434 ) ;
#8925=DIRECTION ( 'NONE',  ( -0.000000000000000000, -0.000000000000000000, -1.000000000000000000 ) ) ;
#8944=FACE_OUTER_BOUND ( 'NONE', #1517, .T. ) ;
#8958=CYLINDRICAL_SURFACE ( 'NONE', #2198, 1.249999999999993339 ) ;
#8960=CARTESIAN_POINT ( 'NONE',  ( 0.000000000000000000, -19.00000000000000711, 0.000000000000000000 ) ) ;
#8976=CARTESIAN_POINT ( 'NONE',  ( 5.999999999999999112, -27.00000000000000711, -4.000000000000000000 ) ) ;
#8986=ORIENTED_EDGE ( 'NONE', *, *, #6749, .T. ) ;
#9009=EDGE_CURVE ( 'NONE', #3093, #9761, #6323, .T. ) ;
#9016=CARTESIAN_POINT ( 'NONE',  ( 0.000000000000000000, 18.99999999999999289, 0.000000000000000000 ) ) ;
#9052=SURFACE_STYLE_USAGE ( .BOTH. , #8051 ) ;
#9055=CARTESIAN_POINT ( 'NONE',  ( 0.000000000000000000, 26.99999999999999289, 1.249999999999988898 ) ) ;
#9059=MECHANICAL_DESIGN_GEOMETRIC_PRESENTATION_REPRESENTATION('',(#1776),#6172);
#9107=LINE ( 'NONE', #9963, #8141 ) ;
#9108=ORIENTED_EDGE ( 'NONE', *, *, #10280, .F. ) ;
#9129=FACE_OUTER_BOUND ( 'NONE', #1410, .T. ) ;
#9140=CARTESIAN_POINT ( 'NONE',  ( 0.000000000000000000, 0.000000000000000000, -4.000000000000000000 ) ) ;
#9141=DIRECTION ( 'NONE',  ( -1.000000000000000000, 0.000000000000000000, 0.000000000000000000 ) ) ;
#9145=FILL_AREA_STYLE ('',( #5997 ) ) ;
#9232=PRODUCT_DEFINITION_FORMATION_WITH_SPECIFIED_SOURCE ( 'ANY', '', #9714, .NOT_KNOWN. ) ;
#9233=DIRECTION ( 'NONE',  ( -0.000000000000000000, -1.000000000000000000, -0.000000000000000000 ) ) ;
#9259=APPLICATION_CONTEXT ( 'automotive_design' ) ;
#9273=CARTESIAN_POINT ( 'NONE',  ( 0.000000000000000000, -27.00000000000000711, 0.000000000000000000 ) ) ;
#9275=CARTESIAN_POINT ( 'NONE',  ( -2.500000000000000000, 0.000000000000000000, 3.000000000000000000 ) ) ;
#9293=ORIENTED_EDGE ( 'NONE', *, *, #9009, .T. ) ;
#9296=DIRECTION ( 'NONE',  ( -0.000000000000000000, 1.000000000000000000, -0.000000000000000000 ) ) ;
#9353=DIRECTION ( 'NONE',  ( -1.000000000000000000, 0.000000000000000000, 0.000000000000000000 ) ) ;
#9365=EDGE_CURVE ( 'NONE', #7779, #144, #5549, .T. ) ;
#9376=EDGE_LOOP ( 'NONE', ( #7074, #7247, #4019 ) ) ;
#9436=LINE ( 'NONE', #5288, #4832 ) ;
#9459=CARTESIAN_POINT ( 'NONE',  ( 0.000000000000000000, 26.99999999999999289, 1.249999999999993339 ) ) ;
#9462=ORIENTED_EDGE ( 'NONE', *, *, #2498, .T. ) ;
#9499=LINE ( 'NONE', #1428, #10409 ) ;
#9506=AXIS2_PLACEMENT_3D ( 'NONE', #4840, #8925, #6533 ) ;
#9527=ORIENTED_EDGE ( 'NONE', *, *, #4025, .F. ) ;
#9539=ORIENTED_EDGE ( 'NONE', *, *, #4965, .F. ) ;
#9556=DIRECTION ( 'NONE',  ( 0.000000000000000000, 0.000000000000000000, -1.000000000000000000 ) ) ;
#9570=EDGE_LOOP ( 'NONE', ( #3067, #4847, #555, #2059 ) ) ;
#9571=DIRECTION ( 'NONE',  ( -0.000000000000000000, -1.000000000000000000, -0.000000000000000000 ) ) ;
#9591=AXIS2_PLACEMENT_3D ( 'NONE', #7645, #968, #7848 ) ;
#9595=DIRECTION ( 'NONE',  ( -0.000000000000000000, -1.000000000000000000, -0.000000000000000000 ) ) ;
#9616=CARTESIAN_POINT ( 'NONE',  ( 5.999999999999999112, 26.99999999999999289, 3.000000000000000000 ) ) ;
#9639=FACE_OUTER_BOUND ( 'NONE', #7012, .T. ) ;
#9646=CARTESIAN_POINT ( 'NONE',  ( -5.999999999999999112, -27.00000000000000711, -4.000000000000000000 ) ) ;
#9664=DIRECTION ( 'NONE',  ( -0.000000000000000000, 1.000000000000000000, -0.000000000000000000 ) ) ;
#9677=AXIS2_PLACEMENT_3D ( 'NONE', #9616, #3242, #5716 ) ;
#9678=EDGE_CURVE ( 'NONE', #10224, #3169, #7455, .T. ) ;
#9686=CARTESIAN_POINT ( 'NONE',  ( -5.999999999999999112, -27.00000000000000711, 3.000000000000000000 ) ) ;
#9714=PRODUCT ( 'cover', 'cover', '', ( #3246 ) ) ;
#9716=DIRECTION ( 'NONE',  ( 1.000000000000000000, 0.000000000000000000, 0.000000000000000000 ) ) ;
#9733=CYLINDRICAL_SURFACE ( 'NONE', #9506, 2.500000000000000000 ) ;
#9761=VERTEX_POINT ( 'NONE', #6537 ) ;
#9789=ORIENTED_EDGE ( 'NONE', *, *, #6082, .T. ) ;
#9801=ORIENTED_EDGE ( 'NONE', *, *, #7995, .T. ) ;
#9814=EDGE_CURVE ( 'NONE', #4115, #7985, #6479, .T. ) ;
#9816=CARTESIAN_POINT ( 'NONE',  ( 0.000000000000000000, 18.99999999999999289, 1.249999999999997558 ) ) ;
#9842=DIRECTION ( 'NONE',  ( 0.000000000000000000, 0.000000000000000000, 1.000000000000000000 ) ) ;
#9930=VERTEX_POINT ( 'NONE', #3085 ) ;
#9950=CARTESIAN_POINT ( 'NONE',  ( 5.999999999999999112, 26.99999999999999289, 3.000000000000000000 ) ) ;
#9963=CARTESIAN_POINT ( 'NONE',  ( 5.999999999999999112, 26.99999999999999289, 3.000000000000000000 ) ) ;
#9975=DIRECTION ( 'NONE',  ( 0.000000000000000000, 0.000000000000000000, -1.000000000000000000 ) ) ;
#9989=CARTESIAN_POINT ( 'NONE',  ( 0.000000000000000000, 26.99999999999999289, 0.000000000000000000 ) ) ;
#10011=CIRCLE ( 'NONE', #5091, 2.500000000000000000 ) ;
#10176=ORIENTED_EDGE ( 'NONE', *, *, #7995, .F. ) ;
#10224=VERTEX_POINT ( 'NONE', #1760 ) ;
#10258=CARTESIAN_POINT ( 'NONE',  ( 5.999999999999999112, 26.99999999999999289, -4.000000000000000000 ) ) ;
#10280=EDGE_CURVE ( 'NONE', #7779, #1248, #479, .T. ) ;
#10286=DIRECTION ( 'NONE',  ( 0.000000000000000000, 0.000000000000000000, -1.000000000000000000 ) ) ;
#10306=LINE ( 'NONE', #9459, #2889 ) ;
#10322=DIRECTION ( 'NONE',  ( -1.000000000000000000, 0.000000000000000000, 0.000000000000000000 ) ) ;
#10333=CONICAL_SURFACE ( 'NONE', #3718, 1.249999999999997558, 1.029744258676650981 ) ;
#10360=AXIS2_PLACEMENT_3D ( 'NONE', #10368, #9296, #4 ) ;
#10368=CARTESIAN_POINT ( 'NONE',  ( 0.000000000000000000, 18.99999999999999289, 0.000000000000000000 ) ) ;
#10395=EDGE_CURVE ( 'NONE', #3169, #4115, #9499, .T. ) ;
#10409=VECTOR ( 'NONE', #8010, 1000.000000000000000 ) ;
#10415=AXIS2_PLACEMENT_3D ( 'NONE', #3751, #3857, #10286 ) ;
#10456=ORIENTED_EDGE ( 'NONE', *, *, #6295, .T. ) ;
#10462=VERTEX_POINT ( 'NONE', #2332 ) ;
#10464=FACE_OUTER_BOUND ( 'NONE', #7731, .T. ) ;
ENDSEC;
END-ISO-10303-21;
